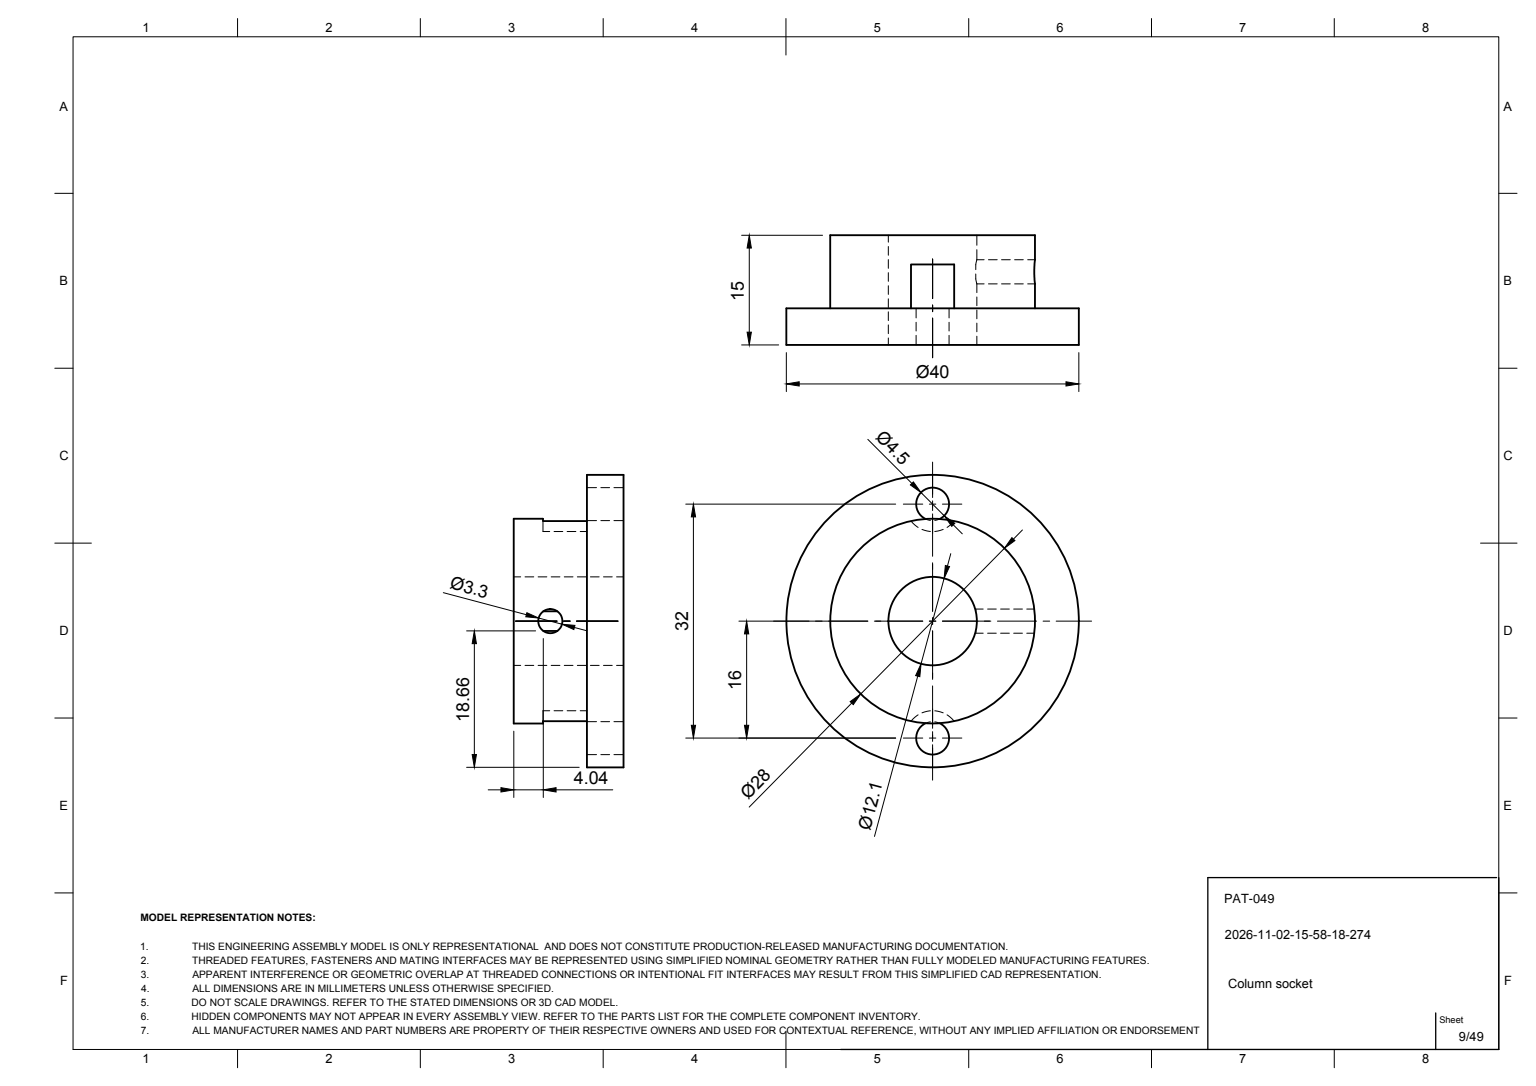
ISO-10303-21;
HEADER;
/* Generated by software containing ST-Developer
 * from STEP Tools, Inc. (www.steptools.com) 
 */

FILE_DESCRIPTION(
/* description */ ('Hand drill press frame (manual)'),
/* implementation_level */ '2;1');

FILE_NAME(
/* name */ 'Column socket.step',
/* time_stamp */ '2026-10-28T03:25:28-07:00',
/* author */ (''),
/* organization */ (''),
/* preprocessor_version */ 'ST-DEVELOPER v20.2',
/* originating_system */ 'Autodesk Translation Framework v15.17.0.0',
/* authorisation */ '');

FILE_SCHEMA (('AUTOMOTIVE_DESIGN { 1 0 10303 214 3 1 1 }'));
ENDSEC;

DATA;
#10=MECHANICAL_DESIGN_GEOMETRIC_PRESENTATION_REPRESENTATION('',(#623),#33299);
#496=B_SPLINE_CURVE_WITH_KNOTS('',3,(#18304,#18305,#18306,#18307,#18308,
#18309,#18310,#18311,#18312,#18313,#18314,#18315,#18316,#18317),
 .UNSPECIFIED.,.F.,.F.,(4,2,2,2,2,2,4),(0.598759573717651,0.624973342427791,
0.687463163426144,0.749952984424497,0.812442805422849,0.874932626421202,
0.901146395131342),.UNSPECIFIED.);
#497=B_SPLINE_CURVE_WITH_KNOTS('',3,(#18321,#18322,#18323,#18324,#18325,
#18326,#18327,#18328),.UNSPECIFIED.,.F.,.F.,(4,2,2,4),(0.249984328141499,
0.312474149139851,0.374963970138204,0.401177738848344),.UNSPECIFIED.);
#498=B_SPLINE_CURVE_WITH_KNOTS('',3,(#18332,#18333,#18334,#18335,#18336,
#18337,#18338,#18339,#18340,#18341,#18342,#18343,#18344,#18345,#18346,#18347,
#18348,#18349,#18350,#18351,#18352,#18353,#18354,#18355,#18356,#18357),
 .UNSPECIFIED.,.F.,.F.,(4,2,2,2,2,2,2,2,2,2,2,2,4),(0.,0.0622156192199746,
0.124431238439949,0.186646447577113,0.248861656714278,0.311076865851442,
0.373292074988606,0.43550769420858,0.497723313428555,0.55993893264853,0.622154551868504,
0.684369761005668,0.746584970142833),.UNSPECIFIED.);
#499=B_SPLINE_CURVE_WITH_KNOTS('',3,(#18358,#18359,#18360,#18361,#18362,
#18363,#18364,#18365,#18366,#18367),.UNSPECIFIED.,.F.,.F.,(4,2,2,2,4),(0.746584970142833,
0.808800179279997,0.871015388417161,0.933231007637136,0.99544662685711),
 .UNSPECIFIED.);
#500=B_SPLINE_CURVE_WITH_KNOTS('',3,(#18368,#18369,#18370,#18371,#18372,
#18373,#18374,#18375),.UNSPECIFIED.,.F.,.F.,(4,2,2,4),(0.0987909174346533,
0.125004686144794,0.187494507143146,0.249984328141499),.UNSPECIFIED.);
#533=SHAPE_REPRESENTATION_RELATIONSHIP('SRR','None',#33492,#578);
#578=ADVANCED_BREP_SHAPE_REPRESENTATION('',(#675),#33254);
#623=STYLED_ITEM('',(#33828),#675);
#675=MANIFOLD_SOLID_BREP('Body1',#12641);
#740=FACE_BOUND('',#2116,.T.);
#741=FACE_BOUND('',#2117,.T.);
#742=FACE_BOUND('',#2118,.T.);
#743=FACE_BOUND('',#2125,.T.);
#744=FACE_BOUND('',#2127,.T.);
#745=FACE_BOUND('',#2129,.T.);
#746=FACE_BOUND('',#2132,.T.);
#747=FACE_BOUND('',#2133,.T.);
#748=FACE_BOUND('',#2134,.T.);
#931=PLANE('',#13301);
#932=PLANE('',#13306);
#933=PLANE('',#13308);
#934=PLANE('',#13315);
#935=PLANE('',#13319);
#936=PLANE('',#13326);
#937=PLANE('',#13332);
#1402=FACE_OUTER_BOUND('',#2111,.T.);
#1403=FACE_OUTER_BOUND('',#2112,.T.);
#1404=FACE_OUTER_BOUND('',#2113,.T.);
#1405=FACE_OUTER_BOUND('',#2114,.T.);
#1406=FACE_OUTER_BOUND('',#2115,.T.);
#1407=FACE_OUTER_BOUND('',#2119,.T.);
#1408=FACE_OUTER_BOUND('',#2120,.T.);
#1409=FACE_OUTER_BOUND('',#2121,.T.);
#1410=FACE_OUTER_BOUND('',#2122,.T.);
#1411=FACE_OUTER_BOUND('',#2123,.T.);
#1412=FACE_OUTER_BOUND('',#2124,.T.);
#1413=FACE_OUTER_BOUND('',#2126,.T.);
#1414=FACE_OUTER_BOUND('',#2128,.T.);
#1415=FACE_OUTER_BOUND('',#2130,.T.);
#1416=FACE_OUTER_BOUND('',#2131,.T.);
#2111=EDGE_LOOP('',(#8713,#8714,#8715,#8716));
#2112=EDGE_LOOP('',(#8717,#8718));
#2113=EDGE_LOOP('',(#8719,#8720,#8721,#8722));
#2114=EDGE_LOOP('',(#8723,#8724));
#2115=EDGE_LOOP('',(#8725));
#2116=EDGE_LOOP('',(#8726,#8727,#8728,#8729,#8730));
#2117=EDGE_LOOP('',(#8731));
#2118=EDGE_LOOP('',(#8732));
#2119=EDGE_LOOP('',(#8733,#8734));
#2120=EDGE_LOOP('',(#8735,#8736,#8737,#8738,#8739,#8740,#8741,#8742,#8743));
#2121=EDGE_LOOP('',(#8744,#8745));
#2122=EDGE_LOOP('',(#8746,#8747,#8748,#8749));
#2123=EDGE_LOOP('',(#8750,#8751,#8752,#8753));
#2124=EDGE_LOOP('',(#8754,#8755,#8756,#8757,#8758,#8759,#8760,#8761,#8762,
#8763,#8764,#8765));
#2125=EDGE_LOOP('',(#8766,#8767));
#2126=EDGE_LOOP('',(#8768));
#2127=EDGE_LOOP('',(#8769));
#2128=EDGE_LOOP('',(#8770,#8771,#8772,#8773));
#2129=EDGE_LOOP('',(#8774,#8775,#8776,#8777,#8778));
#2130=EDGE_LOOP('',(#8779,#8780,#8781,#8782));
#2131=EDGE_LOOP('',(#8783));
#2132=EDGE_LOOP('',(#8784));
#2133=EDGE_LOOP('',(#8785));
#2134=EDGE_LOOP('',(#8786));
#2985=LINE('',#18267,#4150);
#2986=LINE('',#18271,#4151);
#2987=LINE('',#18278,#4152);
#2988=LINE('',#18282,#4153);
#2989=LINE('',#18300,#4154);
#2990=LINE('',#18330,#4155);
#2991=LINE('',#18377,#4156);
#2992=LINE('',#18381,#4157);
#2993=LINE('',#18385,#4158);
#2994=LINE('',#18389,#4159);
#2995=LINE('',#18395,#4160);
#2996=LINE('',#18399,#4161);
#4150=VECTOR('',#14690,1.);
#4151=VECTOR('',#14693,1.);
#4152=VECTOR('',#14702,1.);
#4153=VECTOR('',#14705,1.);
#4154=VECTOR('',#14728,1.);
#4155=VECTOR('',#14735,0.165);
#4156=VECTOR('',#14738,1.);
#4157=VECTOR('',#14743,0.225);
#4158=VECTOR('',#14748,0.225);
#4159=VECTOR('',#14753,1.4);
#4160=VECTOR('',#14760,0.605);
#4161=VECTOR('',#14765,2.);
#5254=CIRCLE('',#13299,0.375);
#5255=CIRCLE('',#13300,0.375);
#5256=CIRCLE('',#13302,1.4);
#5257=CIRCLE('',#13304,0.375);
#5258=CIRCLE('',#13305,0.375);
#5259=CIRCLE('',#13307,1.4);
#5260=CIRCLE('',#13309,2.);
#5261=CIRCLE('',#13310,1.4);
#5262=CIRCLE('',#13311,1.4);
#5263=CIRCLE('',#13312,1.4);
#5264=CIRCLE('',#13313,0.225);
#5265=CIRCLE('',#13314,0.225);
#5266=CIRCLE('',#13316,0.165);
#5267=CIRCLE('',#13318,0.165);
#5268=CIRCLE('',#13321,0.225);
#5269=CIRCLE('',#13323,0.225);
#5270=CIRCLE('',#13325,1.4);
#5271=CIRCLE('',#13327,0.605);
#5272=CIRCLE('',#13329,0.605);
#5273=CIRCLE('',#13331,2.);
#5710=VERTEX_POINT('',#18265);
#5711=VERTEX_POINT('',#18266);
#5712=VERTEX_POINT('',#18268);
#5713=VERTEX_POINT('',#18270);
#5714=VERTEX_POINT('',#18276);
#5715=VERTEX_POINT('',#18277);
#5716=VERTEX_POINT('',#18279);
#5717=VERTEX_POINT('',#18281);
#5718=VERTEX_POINT('',#18287);
#5719=VERTEX_POINT('',#18289);
#5720=VERTEX_POINT('',#18293);
#5721=VERTEX_POINT('',#18295);
#5722=VERTEX_POINT('',#18298);
#5723=VERTEX_POINT('',#18299);
#5724=VERTEX_POINT('',#18303);
#5725=VERTEX_POINT('',#18318);
#5726=VERTEX_POINT('',#18320);
#5727=VERTEX_POINT('',#18329);
#5728=VERTEX_POINT('',#18331);
#5729=VERTEX_POINT('',#18379);
#5730=VERTEX_POINT('',#18383);
#5731=VERTEX_POINT('',#18387);
#5732=VERTEX_POINT('',#18391);
#5733=VERTEX_POINT('',#18394);
#5734=VERTEX_POINT('',#18398);
#6885=EDGE_CURVE('',#5710,#5711,#2985,.T.);
#6886=EDGE_CURVE('',#5710,#5712,#5254,.T.);
#6887=EDGE_CURVE('',#5713,#5712,#2986,.T.);
#6888=EDGE_CURVE('',#5711,#5713,#5255,.T.);
#6889=EDGE_CURVE('',#5712,#5710,#5256,.T.);
#6890=EDGE_CURVE('',#5714,#5715,#2987,.T.);
#6891=EDGE_CURVE('',#5714,#5716,#5257,.T.);
#6892=EDGE_CURVE('',#5717,#5716,#2988,.T.);
#6893=EDGE_CURVE('',#5715,#5717,#5258,.T.);
#6894=EDGE_CURVE('',#5716,#5714,#5259,.T.);
#6895=EDGE_CURVE('',#5718,#5718,#5260,.T.);
#6896=EDGE_CURVE('',#5713,#5719,#5261,.T.);
#6897=EDGE_CURVE('',#5719,#5715,#5262,.T.);
#6898=EDGE_CURVE('',#5717,#5711,#5263,.T.);
#6899=EDGE_CURVE('',#5720,#5720,#5264,.T.);
#6900=EDGE_CURVE('',#5721,#5721,#5265,.T.);
#6901=EDGE_CURVE('',#5722,#5723,#2989,.T.);
#6902=EDGE_CURVE('',#5722,#5723,#5266,.T.);
#6903=EDGE_CURVE('',#5724,#5722,#496,.T.);
#6904=EDGE_CURVE('',#5725,#5724,#5267,.T.);
#6905=EDGE_CURVE('',#5726,#5725,#497,.T.);
#6906=EDGE_CURVE('',#5726,#5727,#2990,.T.);
#6907=EDGE_CURVE('',#5728,#5727,#498,.T.);
#6908=EDGE_CURVE('',#5727,#5728,#499,.T.);
#6909=EDGE_CURVE('',#5723,#5726,#500,.T.);
#6910=EDGE_CURVE('',#5725,#5724,#2991,.T.);
#6911=EDGE_CURVE('',#5729,#5729,#5268,.T.);
#6912=EDGE_CURVE('',#5729,#5720,#2992,.T.);
#6913=EDGE_CURVE('',#5730,#5730,#5269,.T.);
#6914=EDGE_CURVE('',#5730,#5721,#2993,.T.);
#6915=EDGE_CURVE('',#5731,#5731,#5270,.T.);
#6916=EDGE_CURVE('',#5731,#5719,#2994,.T.);
#6917=EDGE_CURVE('',#5732,#5732,#5271,.T.);
#6918=EDGE_CURVE('',#5732,#5733,#2995,.T.);
#6919=EDGE_CURVE('',#5733,#5733,#5272,.T.);
#6920=EDGE_CURVE('',#5718,#5734,#2996,.T.);
#6921=EDGE_CURVE('',#5734,#5734,#5273,.T.);
#8713=ORIENTED_EDGE('',*,*,#6885,.F.);
#8714=ORIENTED_EDGE('',*,*,#6886,.T.);
#8715=ORIENTED_EDGE('',*,*,#6887,.F.);
#8716=ORIENTED_EDGE('',*,*,#6888,.F.);
#8717=ORIENTED_EDGE('',*,*,#6889,.F.);
#8718=ORIENTED_EDGE('',*,*,#6886,.F.);
#8719=ORIENTED_EDGE('',*,*,#6890,.F.);
#8720=ORIENTED_EDGE('',*,*,#6891,.T.);
#8721=ORIENTED_EDGE('',*,*,#6892,.F.);
#8722=ORIENTED_EDGE('',*,*,#6893,.F.);
#8723=ORIENTED_EDGE('',*,*,#6894,.F.);
#8724=ORIENTED_EDGE('',*,*,#6891,.F.);
#8725=ORIENTED_EDGE('',*,*,#6895,.T.);
#8726=ORIENTED_EDGE('',*,*,#6896,.T.);
#8727=ORIENTED_EDGE('',*,*,#6897,.T.);
#8728=ORIENTED_EDGE('',*,*,#6893,.T.);
#8729=ORIENTED_EDGE('',*,*,#6898,.T.);
#8730=ORIENTED_EDGE('',*,*,#6888,.T.);
#8731=ORIENTED_EDGE('',*,*,#6899,.F.);
#8732=ORIENTED_EDGE('',*,*,#6900,.F.);
#8733=ORIENTED_EDGE('',*,*,#6901,.F.);
#8734=ORIENTED_EDGE('',*,*,#6902,.T.);
#8735=ORIENTED_EDGE('',*,*,#6903,.F.);
#8736=ORIENTED_EDGE('',*,*,#6904,.F.);
#8737=ORIENTED_EDGE('',*,*,#6905,.F.);
#8738=ORIENTED_EDGE('',*,*,#6906,.T.);
#8739=ORIENTED_EDGE('',*,*,#6907,.F.);
#8740=ORIENTED_EDGE('',*,*,#6908,.F.);
#8741=ORIENTED_EDGE('',*,*,#6906,.F.);
#8742=ORIENTED_EDGE('',*,*,#6909,.F.);
#8743=ORIENTED_EDGE('',*,*,#6902,.F.);
#8744=ORIENTED_EDGE('',*,*,#6910,.F.);
#8745=ORIENTED_EDGE('',*,*,#6904,.T.);
#8746=ORIENTED_EDGE('',*,*,#6911,.F.);
#8747=ORIENTED_EDGE('',*,*,#6912,.T.);
#8748=ORIENTED_EDGE('',*,*,#6899,.T.);
#8749=ORIENTED_EDGE('',*,*,#6912,.F.);
#8750=ORIENTED_EDGE('',*,*,#6913,.F.);
#8751=ORIENTED_EDGE('',*,*,#6914,.T.);
#8752=ORIENTED_EDGE('',*,*,#6900,.T.);
#8753=ORIENTED_EDGE('',*,*,#6914,.F.);
#8754=ORIENTED_EDGE('',*,*,#6915,.F.);
#8755=ORIENTED_EDGE('',*,*,#6916,.T.);
#8756=ORIENTED_EDGE('',*,*,#6896,.F.);
#8757=ORIENTED_EDGE('',*,*,#6887,.T.);
#8758=ORIENTED_EDGE('',*,*,#6889,.T.);
#8759=ORIENTED_EDGE('',*,*,#6885,.T.);
#8760=ORIENTED_EDGE('',*,*,#6898,.F.);
#8761=ORIENTED_EDGE('',*,*,#6892,.T.);
#8762=ORIENTED_EDGE('',*,*,#6894,.T.);
#8763=ORIENTED_EDGE('',*,*,#6890,.T.);
#8764=ORIENTED_EDGE('',*,*,#6897,.F.);
#8765=ORIENTED_EDGE('',*,*,#6916,.F.);
#8766=ORIENTED_EDGE('',*,*,#6907,.T.);
#8767=ORIENTED_EDGE('',*,*,#6908,.T.);
#8768=ORIENTED_EDGE('',*,*,#6915,.T.);
#8769=ORIENTED_EDGE('',*,*,#6917,.T.);
#8770=ORIENTED_EDGE('',*,*,#6917,.F.);
#8771=ORIENTED_EDGE('',*,*,#6918,.T.);
#8772=ORIENTED_EDGE('',*,*,#6919,.T.);
#8773=ORIENTED_EDGE('',*,*,#6918,.F.);
#8774=ORIENTED_EDGE('',*,*,#6909,.T.);
#8775=ORIENTED_EDGE('',*,*,#6905,.T.);
#8776=ORIENTED_EDGE('',*,*,#6910,.T.);
#8777=ORIENTED_EDGE('',*,*,#6903,.T.);
#8778=ORIENTED_EDGE('',*,*,#6901,.T.);
#8779=ORIENTED_EDGE('',*,*,#6895,.F.);
#8780=ORIENTED_EDGE('',*,*,#6920,.T.);
#8781=ORIENTED_EDGE('',*,*,#6921,.T.);
#8782=ORIENTED_EDGE('',*,*,#6920,.F.);
#8783=ORIENTED_EDGE('',*,*,#6921,.F.);
#8784=ORIENTED_EDGE('',*,*,#6911,.T.);
#8785=ORIENTED_EDGE('',*,*,#6913,.T.);
#8786=ORIENTED_EDGE('',*,*,#6919,.F.);
#11804=CYLINDRICAL_SURFACE('',#13298,0.375);
#11805=CYLINDRICAL_SURFACE('',#13303,0.375);
#11806=CYLINDRICAL_SURFACE('',#13317,0.165);
#11807=CYLINDRICAL_SURFACE('',#13320,0.225);
#11808=CYLINDRICAL_SURFACE('',#13322,0.225);
#11809=CYLINDRICAL_SURFACE('',#13324,1.4);
#11810=CYLINDRICAL_SURFACE('',#13328,0.605);
#11811=CYLINDRICAL_SURFACE('',#13330,2.);
#12011=ADVANCED_FACE('',(#1402),#11804,.F.);
#12012=ADVANCED_FACE('',(#1403),#931,.F.);
#12013=ADVANCED_FACE('',(#1404),#11805,.F.);
#12014=ADVANCED_FACE('',(#1405),#932,.F.);
#12015=ADVANCED_FACE('',(#1406,#740,#741,#742),#933,.T.);
#12016=ADVANCED_FACE('',(#1407),#934,.T.);
#12017=ADVANCED_FACE('',(#1408),#11806,.F.);
#12018=ADVANCED_FACE('',(#1409),#935,.T.);
#12019=ADVANCED_FACE('',(#1410),#11807,.F.);
#12020=ADVANCED_FACE('',(#1411),#11808,.F.);
#12021=ADVANCED_FACE('',(#1412,#743),#11809,.T.);
#12022=ADVANCED_FACE('',(#1413,#744),#936,.T.);
#12023=ADVANCED_FACE('',(#1414,#745),#11810,.F.);
#12024=ADVANCED_FACE('',(#1415),#11811,.T.);
#12025=ADVANCED_FACE('',(#1416,#746,#747,#748),#937,.F.);
#12641=CLOSED_SHELL('',(#12011,#12012,#12013,#12014,#12015,#12016,#12017,
#12018,#12019,#12020,#12021,#12022,#12023,#12024,#12025));
#13297=AXIS2_PLACEMENT_3D('',#18263,#14686,#14687);
#13298=AXIS2_PLACEMENT_3D('',#18264,#14688,#14689);
#13299=AXIS2_PLACEMENT_3D('',#18269,#14691,#14692);
#13300=AXIS2_PLACEMENT_3D('',#18272,#14694,#14695);
#13301=AXIS2_PLACEMENT_3D('',#18273,#14696,#14697);
#13302=AXIS2_PLACEMENT_3D('',#18274,#14698,#14699);
#13303=AXIS2_PLACEMENT_3D('',#18275,#14700,#14701);
#13304=AXIS2_PLACEMENT_3D('',#18280,#14703,#14704);
#13305=AXIS2_PLACEMENT_3D('',#18283,#14706,#14707);
#13306=AXIS2_PLACEMENT_3D('',#18284,#14708,#14709);
#13307=AXIS2_PLACEMENT_3D('',#18285,#14710,#14711);
#13308=AXIS2_PLACEMENT_3D('',#18286,#14712,#14713);
#13309=AXIS2_PLACEMENT_3D('',#18288,#14714,#14715);
#13310=AXIS2_PLACEMENT_3D('',#18290,#14716,#14717);
#13311=AXIS2_PLACEMENT_3D('',#18291,#14718,#14719);
#13312=AXIS2_PLACEMENT_3D('',#18292,#14720,#14721);
#13313=AXIS2_PLACEMENT_3D('',#18294,#14722,#14723);
#13314=AXIS2_PLACEMENT_3D('',#18296,#14724,#14725);
#13315=AXIS2_PLACEMENT_3D('',#18297,#14726,#14727);
#13316=AXIS2_PLACEMENT_3D('',#18301,#14729,#14730);
#13317=AXIS2_PLACEMENT_3D('',#18302,#14731,#14732);
#13318=AXIS2_PLACEMENT_3D('',#18319,#14733,#14734);
#13319=AXIS2_PLACEMENT_3D('',#18376,#14736,#14737);
#13320=AXIS2_PLACEMENT_3D('',#18378,#14739,#14740);
#13321=AXIS2_PLACEMENT_3D('',#18380,#14741,#14742);
#13322=AXIS2_PLACEMENT_3D('',#18382,#14744,#14745);
#13323=AXIS2_PLACEMENT_3D('',#18384,#14746,#14747);
#13324=AXIS2_PLACEMENT_3D('',#18386,#14749,#14750);
#13325=AXIS2_PLACEMENT_3D('',#18388,#14751,#14752);
#13326=AXIS2_PLACEMENT_3D('',#18390,#14754,#14755);
#13327=AXIS2_PLACEMENT_3D('',#18392,#14756,#14757);
#13328=AXIS2_PLACEMENT_3D('',#18393,#14758,#14759);
#13329=AXIS2_PLACEMENT_3D('',#18396,#14761,#14762);
#13330=AXIS2_PLACEMENT_3D('',#18397,#14763,#14764);
#13331=AXIS2_PLACEMENT_3D('',#18400,#14766,#14767);
#13332=AXIS2_PLACEMENT_3D('',#18401,#14768,#14769);
#14686=DIRECTION('axis',(0.,0.,1.));
#14687=DIRECTION('refdir',(1.,0.,0.));
#14688=DIRECTION('center_axis',(0.,0.,1.));
#14689=DIRECTION('ref_axis',(1.,0.,0.));
#14690=DIRECTION('',(0.,0.,-1.));
#14691=DIRECTION('center_axis',(0.,0.,1.));
#14692=DIRECTION('ref_axis',(1.,0.,0.));
#14693=DIRECTION('',(0.,0.,1.));
#14694=DIRECTION('center_axis',(0.,0.,1.));
#14695=DIRECTION('ref_axis',(1.,0.,0.));
#14696=DIRECTION('center_axis',(0.,0.,1.));
#14697=DIRECTION('ref_axis',(1.,0.,0.));
#14698=DIRECTION('center_axis',(0.,0.,1.));
#14699=DIRECTION('ref_axis',(1.,0.,0.));
#14700=DIRECTION('center_axis',(0.,0.,1.));
#14701=DIRECTION('ref_axis',(1.,0.,0.));
#14702=DIRECTION('',(0.,0.,-1.));
#14703=DIRECTION('center_axis',(0.,0.,1.));
#14704=DIRECTION('ref_axis',(1.,0.,0.));
#14705=DIRECTION('',(0.,0.,1.));
#14706=DIRECTION('center_axis',(0.,0.,1.));
#14707=DIRECTION('ref_axis',(1.,0.,0.));
#14708=DIRECTION('center_axis',(0.,0.,1.));
#14709=DIRECTION('ref_axis',(1.,0.,0.));
#14710=DIRECTION('center_axis',(0.,0.,1.));
#14711=DIRECTION('ref_axis',(1.,0.,0.));
#14712=DIRECTION('center_axis',(0.,0.,1.));
#14713=DIRECTION('ref_axis',(1.,0.,0.));
#14714=DIRECTION('center_axis',(0.,0.,1.));
#14715=DIRECTION('ref_axis',(1.,0.,0.));
#14716=DIRECTION('center_axis',(0.,0.,-1.));
#14717=DIRECTION('ref_axis',(1.,0.,0.));
#14718=DIRECTION('center_axis',(0.,0.,-1.));
#14719=DIRECTION('ref_axis',(1.,0.,0.));
#14720=DIRECTION('center_axis',(0.,0.,-1.));
#14721=DIRECTION('ref_axis',(1.,0.,0.));
#14722=DIRECTION('center_axis',(0.,0.,1.));
#14723=DIRECTION('ref_axis',(1.,0.,0.));
#14724=DIRECTION('center_axis',(0.,0.,1.));
#14725=DIRECTION('ref_axis',(1.,0.,0.));
#14726=DIRECTION('center_axis',(1.,0.,0.));
#14727=DIRECTION('ref_axis',(0.,0.,-1.));
#14728=DIRECTION('',(0.,0.,1.));
#14729=DIRECTION('center_axis',(1.,0.,0.));
#14730=DIRECTION('ref_axis',(0.,0.,-1.));
#14731=DIRECTION('center_axis',(1.,0.,0.));
#14732=DIRECTION('ref_axis',(0.,0.,-1.));
#14733=DIRECTION('center_axis',(1.,0.,0.));
#14734=DIRECTION('ref_axis',(0.,0.,-1.));
#14735=DIRECTION('',(1.,0.,0.));
#14736=DIRECTION('center_axis',(1.,0.,0.));
#14737=DIRECTION('ref_axis',(0.,0.,-1.));
#14738=DIRECTION('',(0.,0.,-1.));
#14739=DIRECTION('center_axis',(0.,0.,1.));
#14740=DIRECTION('ref_axis',(1.,0.,0.));
#14741=DIRECTION('center_axis',(0.,0.,1.));
#14742=DIRECTION('ref_axis',(1.,0.,0.));
#14743=DIRECTION('',(0.,0.,1.));
#14744=DIRECTION('center_axis',(0.,0.,1.));
#14745=DIRECTION('ref_axis',(1.,0.,0.));
#14746=DIRECTION('center_axis',(0.,0.,1.));
#14747=DIRECTION('ref_axis',(1.,0.,0.));
#14748=DIRECTION('',(0.,0.,1.));
#14749=DIRECTION('center_axis',(0.,0.,1.));
#14750=DIRECTION('ref_axis',(1.,0.,0.));
#14751=DIRECTION('center_axis',(0.,0.,1.));
#14752=DIRECTION('ref_axis',(1.,0.,0.));
#14753=DIRECTION('',(0.,0.,-1.));
#14754=DIRECTION('center_axis',(0.,0.,1.));
#14755=DIRECTION('ref_axis',(1.,0.,0.));
#14756=DIRECTION('center_axis',(0.,0.,-1.));
#14757=DIRECTION('ref_axis',(1.,0.,0.));
#14758=DIRECTION('center_axis',(0.,0.,1.));
#14759=DIRECTION('ref_axis',(1.,0.,0.));
#14760=DIRECTION('',(0.,0.,-1.));
#14761=DIRECTION('center_axis',(0.,0.,-1.));
#14762=DIRECTION('ref_axis',(1.,0.,0.));
#14763=DIRECTION('center_axis',(0.,0.,1.));
#14764=DIRECTION('ref_axis',(1.,0.,0.));
#14765=DIRECTION('',(0.,0.,-1.));
#14766=DIRECTION('center_axis',(0.,0.,1.));
#14767=DIRECTION('ref_axis',(1.,0.,0.));
#14768=DIRECTION('center_axis',(0.,0.,1.));
#14769=DIRECTION('ref_axis',(1.,0.,0.));
#18263=CARTESIAN_POINT('',(0.,0.,0.));
#18264=CARTESIAN_POINT('Origin',(5.5,-1.6,1.5));
#18265=CARTESIAN_POINT('',(5.79505604098506,-1.3685546875,2.1));
#18266=CARTESIAN_POINT('',(5.79505604098506,-1.3685546875,1.5));
#18267=CARTESIAN_POINT('',(5.79505604098506,-1.3685546875,1.5));
#18268=CARTESIAN_POINT('',(5.20494395901494,-1.3685546875,2.1));
#18269=CARTESIAN_POINT('Origin',(5.5,-1.6,2.1));
#18270=CARTESIAN_POINT('',(5.20494395901494,-1.3685546875,1.5));
#18271=CARTESIAN_POINT('',(5.20494395901494,-1.3685546875,1.5));
#18272=CARTESIAN_POINT('Origin',(5.5,-1.6,1.5));
#18273=CARTESIAN_POINT('Origin',(5.5,-1.6,2.1));
#18274=CARTESIAN_POINT('Origin',(5.5,0.,2.1));
#18275=CARTESIAN_POINT('Origin',(5.5,1.6,1.5));
#18276=CARTESIAN_POINT('',(5.20494395901494,1.3685546875,2.1));
#18277=CARTESIAN_POINT('',(5.20494395901494,1.3685546875,1.5));
#18278=CARTESIAN_POINT('',(5.20494395901494,1.3685546875,1.5));
#18279=CARTESIAN_POINT('',(5.79505604098506,1.3685546875,2.1));
#18280=CARTESIAN_POINT('Origin',(5.5,1.6,2.1));
#18281=CARTESIAN_POINT('',(5.79505604098506,1.3685546875,1.5));
#18282=CARTESIAN_POINT('',(5.79505604098506,1.3685546875,1.5));
#18283=CARTESIAN_POINT('Origin',(5.5,1.6,1.5));
#18284=CARTESIAN_POINT('Origin',(5.5,1.6,2.1));
#18285=CARTESIAN_POINT('Origin',(5.5,0.,2.1));
#18286=CARTESIAN_POINT('Origin',(5.5,0.,1.5));
#18287=CARTESIAN_POINT('',(3.5,-2.44929359829471E-16,1.5));
#18288=CARTESIAN_POINT('Origin',(5.5,0.,1.5));
#18289=CARTESIAN_POINT('',(4.1,-1.71450551880629E-16,1.5));
#18290=CARTESIAN_POINT('Origin',(5.5,0.,1.5));
#18291=CARTESIAN_POINT('Origin',(5.5,0.,1.5));
#18292=CARTESIAN_POINT('Origin',(5.5,0.,1.5));
#18293=CARTESIAN_POINT('',(5.275,-1.6,1.5));
#18294=CARTESIAN_POINT('Origin',(5.5,-1.6,1.5));
#18295=CARTESIAN_POINT('',(5.275,1.6,1.5));
#18296=CARTESIAN_POINT('Origin',(5.5,1.6,1.5));
#18297=CARTESIAN_POINT('Origin',(6.09,0.,2.));
#18298=CARTESIAN_POINT('',(6.09,0.133884278389961,1.90356349239007));
#18299=CARTESIAN_POINT('',(6.09,0.133884278389961,2.09643650760993));
#18300=CARTESIAN_POINT('',(6.09,0.133884278389961,1.));
#18301=CARTESIAN_POINT('Origin',(6.09,0.,2.));
#18302=CARTESIAN_POINT('Origin',(6.09,0.,2.));
#18303=CARTESIAN_POINT('',(6.09,-0.133884278389961,1.90356349239007));
#18304=CARTESIAN_POINT('Ctrl Pts',(6.09,-0.133884278389961,1.90356349239007));
#18305=CARTESIAN_POINT('Ctrl Pts',(6.09119840340611,-0.128603165341395,
1.89623164237677));
#18306=CARTESIAN_POINT('Ctrl Pts',(6.09244064128815,-0.122792448979944,
1.88944721118838));
#18307=CARTESIAN_POINT('Ctrl Pts',(6.09651064111414,-0.10208383195986,1.8687385941683));
#18308=CARTESIAN_POINT('Ctrl Pts',(6.09954409498317,-0.0836002135946606,
1.8560565239921));
#18309=CARTESIAN_POINT('Ctrl Pts',(6.10381707438298,-0.0429774150042654,
1.8391843843662));
#18310=CARTESIAN_POINT('Ctrl Pts',(6.105,-0.0208299403327843,1.835));
#18311=CARTESIAN_POINT('Ctrl Pts',(6.105,0.0208299403327842,1.835));
#18312=CARTESIAN_POINT('Ctrl Pts',(6.10381707438298,0.0429774150042654,
1.8391843843662));
#18313=CARTESIAN_POINT('Ctrl Pts',(6.09954409498317,0.0836002135946606,
1.8560565239921));
#18314=CARTESIAN_POINT('Ctrl Pts',(6.09651064111414,0.10208383195986,1.8687385941683));
#18315=CARTESIAN_POINT('Ctrl Pts',(6.09244064128815,0.122792448979944,1.88944721118838));
#18316=CARTESIAN_POINT('Ctrl Pts',(6.09119840340611,0.128603165341395,1.89623164237677));
#18317=CARTESIAN_POINT('Ctrl Pts',(6.09,0.133884278389961,1.90356349239007));
#18318=CARTESIAN_POINT('',(6.09,-0.133884278389961,2.09643650760993));
#18319=CARTESIAN_POINT('Origin',(6.09,0.,2.));
#18320=CARTESIAN_POINT('',(6.105,-3.4389464756641E-17,2.165));
#18321=CARTESIAN_POINT('Ctrl Pts',(6.105,-4.85722573273506E-17,2.165));
#18322=CARTESIAN_POINT('Ctrl Pts',(6.105,-0.0208299403327842,2.165));
#18323=CARTESIAN_POINT('Ctrl Pts',(6.10381707438298,-0.0429774150042653,
2.1608156156338));
#18324=CARTESIAN_POINT('Ctrl Pts',(6.09954409498317,-0.0836002135946605,
2.1439434760079));
#18325=CARTESIAN_POINT('Ctrl Pts',(6.09651064111414,-0.10208383195986,2.1312614058317));
#18326=CARTESIAN_POINT('Ctrl Pts',(6.09244064128815,-0.122792448979944,
2.11055278881162));
#18327=CARTESIAN_POINT('Ctrl Pts',(6.09119840340611,-0.128603165341395,
2.10376835762323));
#18328=CARTESIAN_POINT('Ctrl Pts',(6.09,-0.133884278389961,2.09643650760993));
#18329=CARTESIAN_POINT('',(6.9,-2.02066721859313E-17,2.165));
#18330=CARTESIAN_POINT('',(6.09,-2.02066721859313E-17,2.165));
#18331=CARTESIAN_POINT('',(6.8902427845524,0.165,2.));
#18332=CARTESIAN_POINT('Ctrl Pts',(6.8902427845524,0.165,2.));
#18333=CARTESIAN_POINT('Ctrl Pts',(6.8902427845524,0.165,1.97926146026001));
#18334=CARTESIAN_POINT('Ctrl Pts',(6.89075468722975,0.16085144747456,1.95715388604164));
#18335=CARTESIAN_POINT('Ctrl Pts',(6.89259968365095,0.144006627864301,1.9165070705051));
#18336=CARTESIAN_POINT('Ctrl Pts',(6.89390570229761,0.131311408395222,1.89796617060366));
#18337=CARTESIAN_POINT('Ctrl Pts',(6.89635413416378,0.102033925885227,1.86868868809367));
#18338=CARTESIAN_POINT('Ctrl Pts',(6.89765618378145,0.0834929839417279,
1.85599339308932));
#18339=CARTESIAN_POINT('Ctrl Pts',(6.89949208802221,0.0428460264460561,
1.83914851786885));
#18340=CARTESIAN_POINT('Ctrl Pts',(6.9,0.0207384030457214,1.835));
#18341=CARTESIAN_POINT('Ctrl Pts',(6.9,-0.0207384030457214,1.835));
#18342=CARTESIAN_POINT('Ctrl Pts',(6.89949208802221,-0.042846026446056,
1.83914851786885));
#18343=CARTESIAN_POINT('Ctrl Pts',(6.89765618378145,-0.0834929839417279,
1.85599339308932));
#18344=CARTESIAN_POINT('Ctrl Pts',(6.89635413416378,-0.102033925885227,
1.86868868809367));
#18345=CARTESIAN_POINT('Ctrl Pts',(6.89390570229761,-0.131311408395222,
1.89796617060366));
#18346=CARTESIAN_POINT('Ctrl Pts',(6.89259968365095,-0.144006627864301,
1.9165070705051));
#18347=CARTESIAN_POINT('Ctrl Pts',(6.89075468722975,-0.16085144747456,1.95715388604164));
#18348=CARTESIAN_POINT('Ctrl Pts',(6.8902427845524,-0.165,1.97926146026001));
#18349=CARTESIAN_POINT('Ctrl Pts',(6.8902427845524,-0.165,2.02073853973999));
#18350=CARTESIAN_POINT('Ctrl Pts',(6.89075468722975,-0.160851447474559,
2.04284611395836));
#18351=CARTESIAN_POINT('Ctrl Pts',(6.89259968365095,-0.144006627864301,
2.0834929294949));
#18352=CARTESIAN_POINT('Ctrl Pts',(6.89390570229761,-0.131311408395222,
2.10203382939634));
#18353=CARTESIAN_POINT('Ctrl Pts',(6.89635413416378,-0.102033925885227,
2.13131131190633));
#18354=CARTESIAN_POINT('Ctrl Pts',(6.89765618378145,-0.0834929839417278,
2.14400660691068));
#18355=CARTESIAN_POINT('Ctrl Pts',(6.89949208802221,-0.0428460264460559,
2.16085148213115));
#18356=CARTESIAN_POINT('Ctrl Pts',(6.9,-0.0207384030457214,2.165));
#18357=CARTESIAN_POINT('Ctrl Pts',(6.9,-6.24500451351651E-17,2.165));
#18358=CARTESIAN_POINT('Ctrl Pts',(6.9,-2.42861286636753E-17,2.165));
#18359=CARTESIAN_POINT('Ctrl Pts',(6.9,0.0207384030457214,2.165));
#18360=CARTESIAN_POINT('Ctrl Pts',(6.89949208802221,0.0428460264460559,
2.16085148213115));
#18361=CARTESIAN_POINT('Ctrl Pts',(6.89765618378145,0.0834929839417279,
2.14400660691068));
#18362=CARTESIAN_POINT('Ctrl Pts',(6.89635413416378,0.102033925885227,2.13131131190633));
#18363=CARTESIAN_POINT('Ctrl Pts',(6.89390570229761,0.131311408395222,2.10203382939634));
#18364=CARTESIAN_POINT('Ctrl Pts',(6.89259968365095,0.144006627864301,2.0834929294949));
#18365=CARTESIAN_POINT('Ctrl Pts',(6.89075468722975,0.160851447474559,2.04284611395836));
#18366=CARTESIAN_POINT('Ctrl Pts',(6.8902427845524,0.165,2.02073853973999));
#18367=CARTESIAN_POINT('Ctrl Pts',(6.8902427845524,0.165,2.));
#18368=CARTESIAN_POINT('Ctrl Pts',(6.09,0.133884278389961,2.09643650760993));
#18369=CARTESIAN_POINT('Ctrl Pts',(6.09119840340611,0.128603165341395,2.10376835762323));
#18370=CARTESIAN_POINT('Ctrl Pts',(6.09244064128815,0.122792448979944,2.11055278881162));
#18371=CARTESIAN_POINT('Ctrl Pts',(6.09651064111414,0.10208383195986,2.1312614058317));
#18372=CARTESIAN_POINT('Ctrl Pts',(6.09954409498317,0.0836002135946605,
2.1439434760079));
#18373=CARTESIAN_POINT('Ctrl Pts',(6.10381707438298,0.0429774150042653,
2.1608156156338));
#18374=CARTESIAN_POINT('Ctrl Pts',(6.105,0.0208299403327843,2.165));
#18375=CARTESIAN_POINT('Ctrl Pts',(6.105,6.24500451351651E-17,2.165));
#18376=CARTESIAN_POINT('Origin',(6.09,0.,2.));
#18377=CARTESIAN_POINT('',(6.09,-0.133884278389961,1.));
#18378=CARTESIAN_POINT('Origin',(5.5,-1.6,0.9));
#18379=CARTESIAN_POINT('',(5.275,-1.6,1.));
#18380=CARTESIAN_POINT('Origin',(5.5,-1.6,1.));
#18381=CARTESIAN_POINT('',(5.275,-1.6,0.9));
#18382=CARTESIAN_POINT('Origin',(5.5,1.6,0.9));
#18383=CARTESIAN_POINT('',(5.275,1.6,1.));
#18384=CARTESIAN_POINT('Origin',(5.5,1.6,1.));
#18385=CARTESIAN_POINT('',(5.275,1.6,0.9));
#18386=CARTESIAN_POINT('Origin',(5.5,0.,1.5));
#18387=CARTESIAN_POINT('',(4.1,-1.71450551880629E-16,2.5));
#18388=CARTESIAN_POINT('Origin',(5.5,0.,2.5));
#18389=CARTESIAN_POINT('',(4.1,-1.71450551880629E-16,1.5));
#18390=CARTESIAN_POINT('Origin',(5.5,0.,2.5));
#18391=CARTESIAN_POINT('',(4.895,-7.40911313484149E-17,2.5));
#18392=CARTESIAN_POINT('Origin',(5.5,0.,2.5));
#18393=CARTESIAN_POINT('Origin',(5.5,0.,1.));
#18394=CARTESIAN_POINT('',(4.895,-7.40911313484149E-17,1.));
#18395=CARTESIAN_POINT('',(4.895,-7.40911313484149E-17,1.));
#18396=CARTESIAN_POINT('Origin',(5.5,0.,1.));
#18397=CARTESIAN_POINT('Origin',(5.5,0.,1.));
#18398=CARTESIAN_POINT('',(3.5,-2.44929359829471E-16,1.));
#18399=CARTESIAN_POINT('',(3.5,-2.44929359829471E-16,1.));
#18400=CARTESIAN_POINT('Origin',(5.5,0.,1.));
#18401=CARTESIAN_POINT('Origin',(5.5,0.,1.));
#33202=UNCERTAINTY_MEASURE_WITH_UNIT(LENGTH_MEASURE(0.001),#33300,
'DISTANCE_ACCURACY_VALUE',
'Maximum model space distance between geometric entities at asserted c
onnectivities');
#33247=UNCERTAINTY_MEASURE_WITH_UNIT(LENGTH_MEASURE(0.001),#33300,
'DISTANCE_ACCURACY_VALUE',
'Maximum model space distance between geometric entities at asserted c
onnectivities');
#33254=(
GEOMETRIC_REPRESENTATION_CONTEXT(3)
GLOBAL_UNCERTAINTY_ASSIGNED_CONTEXT((#33202))
GLOBAL_UNIT_ASSIGNED_CONTEXT((#33300,#33302,#33303))
REPRESENTATION_CONTEXT('','3D')
);
#33299=(
GEOMETRIC_REPRESENTATION_CONTEXT(3)
GLOBAL_UNCERTAINTY_ASSIGNED_CONTEXT((#33247))
GLOBAL_UNIT_ASSIGNED_CONTEXT((#33300,#33302,#33303))
REPRESENTATION_CONTEXT('','3D')
);
#33300=(
LENGTH_UNIT()
NAMED_UNIT(*)
SI_UNIT(.CENTI.,.METRE.)
);
#33302=(
NAMED_UNIT(*)
PLANE_ANGLE_UNIT()
SI_UNIT($,.RADIAN.)
);
#33303=(
NAMED_UNIT(*)
SI_UNIT($,.STERADIAN.)
SOLID_ANGLE_UNIT()
);
#33310=SHAPE_DEFINITION_REPRESENTATION(#33361,#33492);
#33361=PRODUCT_DEFINITION_SHAPE('',$,#33544);
#33492=SHAPE_REPRESENTATION('',(#13297),#33254);
#33537=PRODUCT_DEFINITION_CONTEXT('part definition',#33692,'design');
#33544=PRODUCT_DEFINITION('Column socket','Column socket',#33595,#33537);
#33595=PRODUCT_DEFINITION_FORMATION('',$,#33700);
#33692=APPLICATION_CONTEXT(
'Core Data for Automotive Mechanical Design Process');
#33693=PRODUCT_CONTEXT('part definition',#33692,'mechanical');
#33700=PRODUCT('Column socket','Column socket','Column socket',(#33693));
#33822=COLOUR_RGB('Off White',0.89,0.88,0.83);
#33823=FILL_AREA_STYLE_COLOUR('',#33822);
#33824=FILL_AREA_STYLE('',(#33823));
#33825=SURFACE_STYLE_FILL_AREA(#33824);
#33826=SURFACE_SIDE_STYLE('',(#33825));
#33827=SURFACE_STYLE_USAGE(.BOTH.,#33826);
#33828=PRESENTATION_STYLE_ASSIGNMENT((#33827));
ENDSEC;
END-ISO-10303-21;
